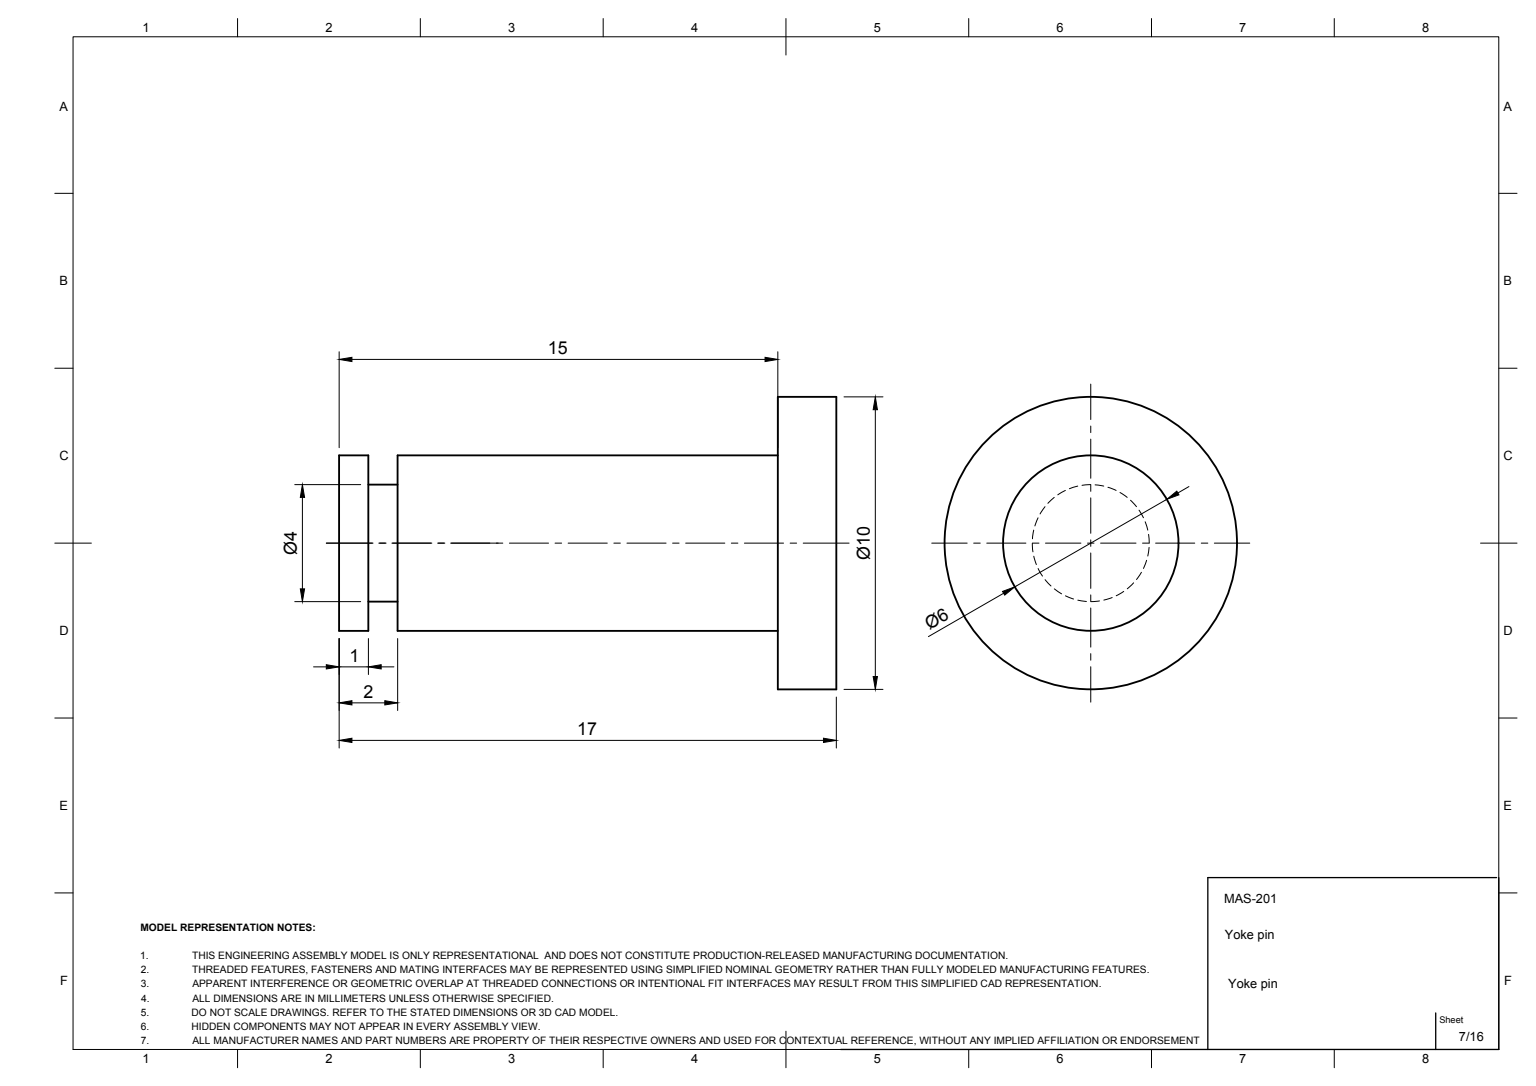
ISO-10303-21;
HEADER;
/* Generated by software containing ST-Developer
 * from STEP Tools, Inc. (www.steptools.com) 
 */

FILE_DESCRIPTION(
/* description */ ('Independent manual two-gate roller-track escapement for nominal30mm d
iameter20mm wide feed rollers. Opposed gates are driven by native capt
ured pin-slot loops with positive curved-slot travel stops at\X\B116de
g. Repeated gate/pin/washer/clip instances, adapted native common bear
ing families, full retaining lips and rotating polymer grip. External 
workpieces, gravity feeder/incline and mount anchors outside assembly.
 No powered-feed compatibility, impact, capacity, safety, force, wear 
or life rating.'),
/* implementation_level */ '2;1');

FILE_NAME(
/* name */ 'Yoke pin.step',
/* time_stamp */ '2026-11-08T18:43:23-08:00',
/* author */ (''),
/* organization */ (''),
/* preprocessor_version */ 'ST-DEVELOPER v20.2',
/* originating_system */ 'Autodesk Translation Framework v15.17.0.0',
/* authorisation */ '');

FILE_SCHEMA (('AUTOMOTIVE_DESIGN { 1 0 10303 214 3 1 1 }'));
ENDSEC;

DATA;
#10=MECHANICAL_DESIGN_GEOMETRIC_PRESENTATION_REPRESENTATION('',(#459),#19863);
#421=SHAPE_REPRESENTATION_RELATIONSHIP('SRR','None',#19939,#440);
#440=ADVANCED_BREP_SHAPE_REPRESENTATION('',(#478),#19848);
#459=STYLED_ITEM('',(#20042),#478);
#478=MANIFOLD_SOLID_BREP('Body1',#6428);
#826=LINE('',#15773,#1291);
#827=LINE('',#15784,#1292);
#828=LINE('',#15792,#1293);
#829=LINE('',#15796,#1294);
#1291=VECTOR('',#8076,2.);
#1292=VECTOR('',#8091,3.);
#1293=VECTOR('',#8100,5.);
#1294=VECTOR('',#8107,3.);
#1536=CYLINDRICAL_SURFACE('',#6927,2.);
#1537=CYLINDRICAL_SURFACE('',#6934,3.);
#1538=CYLINDRICAL_SURFACE('',#6939,5.);
#1539=CYLINDRICAL_SURFACE('',#6942,3.);
#1659=FACE_BOUND('',#2300,.T.);
#1660=FACE_BOUND('',#2302,.T.);
#1661=FACE_BOUND('',#2305,.T.);
#1897=FACE_OUTER_BOUND('',#2298,.T.);
#1898=FACE_OUTER_BOUND('',#2299,.T.);
#1899=FACE_OUTER_BOUND('',#2301,.T.);
#1900=FACE_OUTER_BOUND('',#2303,.T.);
#1901=FACE_OUTER_BOUND('',#2304,.T.);
#1902=FACE_OUTER_BOUND('',#2306,.T.);
#1903=FACE_OUTER_BOUND('',#2307,.T.);
#1904=FACE_OUTER_BOUND('',#2308,.T.);
#1905=FACE_OUTER_BOUND('',#2309,.T.);
#2298=EDGE_LOOP('',(#5289,#5290,#5291,#5292));
#2299=EDGE_LOOP('',(#5293));
#2300=EDGE_LOOP('',(#5294));
#2301=EDGE_LOOP('',(#5295));
#2302=EDGE_LOOP('',(#5296));
#2303=EDGE_LOOP('',(#5297,#5298,#5299,#5300));
#2304=EDGE_LOOP('',(#5301));
#2305=EDGE_LOOP('',(#5302));
#2306=EDGE_LOOP('',(#5303,#5304,#5305,#5306));
#2307=EDGE_LOOP('',(#5307));
#2308=EDGE_LOOP('',(#5308,#5309,#5310,#5311));
#2309=EDGE_LOOP('',(#5312));
#2538=CIRCLE('',#6928,2.);
#2539=CIRCLE('',#6929,2.);
#2540=CIRCLE('',#6931,3.);
#2541=CIRCLE('',#6933,3.);
#2542=CIRCLE('',#6935,3.);
#2543=CIRCLE('',#6937,5.);
#2544=CIRCLE('',#6938,3.);
#2545=CIRCLE('',#6940,5.);
#3008=VERTEX_POINT('',#15770);
#3009=VERTEX_POINT('',#15772);
#3010=VERTEX_POINT('',#15776);
#3011=VERTEX_POINT('',#15779);
#3012=VERTEX_POINT('',#15782);
#3013=VERTEX_POINT('',#15786);
#3014=VERTEX_POINT('',#15788);
#3015=VERTEX_POINT('',#15791);
#3803=EDGE_CURVE('',#3008,#3008,#2538,.T.);
#3804=EDGE_CURVE('',#3008,#3009,#826,.T.);
#3805=EDGE_CURVE('',#3009,#3009,#2539,.T.);
#3806=EDGE_CURVE('',#3010,#3010,#2540,.T.);
#3807=EDGE_CURVE('',#3011,#3011,#2541,.T.);
#3808=EDGE_CURVE('',#3012,#3012,#2542,.T.);
#3809=EDGE_CURVE('',#3012,#3011,#827,.T.);
#3810=EDGE_CURVE('',#3013,#3013,#2543,.T.);
#3811=EDGE_CURVE('',#3014,#3014,#2544,.T.);
#3812=EDGE_CURVE('',#3013,#3015,#828,.T.);
#3813=EDGE_CURVE('',#3015,#3015,#2545,.T.);
#3814=EDGE_CURVE('',#3010,#3014,#829,.T.);
#5289=ORIENTED_EDGE('',*,*,#3803,.T.);
#5290=ORIENTED_EDGE('',*,*,#3804,.T.);
#5291=ORIENTED_EDGE('',*,*,#3805,.F.);
#5292=ORIENTED_EDGE('',*,*,#3804,.F.);
#5293=ORIENTED_EDGE('',*,*,#3806,.F.);
#5294=ORIENTED_EDGE('',*,*,#3803,.F.);
#5295=ORIENTED_EDGE('',*,*,#3807,.F.);
#5296=ORIENTED_EDGE('',*,*,#3805,.T.);
#5297=ORIENTED_EDGE('',*,*,#3808,.F.);
#5298=ORIENTED_EDGE('',*,*,#3809,.T.);
#5299=ORIENTED_EDGE('',*,*,#3807,.T.);
#5300=ORIENTED_EDGE('',*,*,#3809,.F.);
#5301=ORIENTED_EDGE('',*,*,#3810,.T.);
#5302=ORIENTED_EDGE('',*,*,#3811,.F.);
#5303=ORIENTED_EDGE('',*,*,#3810,.F.);
#5304=ORIENTED_EDGE('',*,*,#3812,.T.);
#5305=ORIENTED_EDGE('',*,*,#3813,.T.);
#5306=ORIENTED_EDGE('',*,*,#3812,.F.);
#5307=ORIENTED_EDGE('',*,*,#3813,.F.);
#5308=ORIENTED_EDGE('',*,*,#3806,.T.);
#5309=ORIENTED_EDGE('',*,*,#3814,.T.);
#5310=ORIENTED_EDGE('',*,*,#3811,.T.);
#5311=ORIENTED_EDGE('',*,*,#3814,.F.);
#5312=ORIENTED_EDGE('',*,*,#3808,.T.);
#6004=PLANE('',#6930);
#6005=PLANE('',#6932);
#6006=PLANE('',#6936);
#6007=PLANE('',#6941);
#6008=PLANE('',#6943);
#6276=ADVANCED_FACE('',(#1897),#1536,.T.);
#6277=ADVANCED_FACE('',(#1898,#1659),#6004,.F.);
#6278=ADVANCED_FACE('',(#1899,#1660),#6005,.F.);
#6279=ADVANCED_FACE('',(#1900),#1537,.T.);
#6280=ADVANCED_FACE('',(#1901,#1661),#6006,.T.);
#6281=ADVANCED_FACE('',(#1902),#1538,.T.);
#6282=ADVANCED_FACE('',(#1903),#6007,.F.);
#6283=ADVANCED_FACE('',(#1904),#1539,.T.);
#6284=ADVANCED_FACE('',(#1905),#6008,.T.);
#6428=CLOSED_SHELL('',(#6276,#6277,#6278,#6279,#6280,#6281,#6282,#6283,
#6284));
#6926=AXIS2_PLACEMENT_3D('',#15768,#8070,#8071);
#6927=AXIS2_PLACEMENT_3D('',#15769,#8072,#8073);
#6928=AXIS2_PLACEMENT_3D('',#15771,#8074,#8075);
#6929=AXIS2_PLACEMENT_3D('',#15774,#8077,#8078);
#6930=AXIS2_PLACEMENT_3D('',#15775,#8079,#8080);
#6931=AXIS2_PLACEMENT_3D('',#15777,#8081,#8082);
#6932=AXIS2_PLACEMENT_3D('',#15778,#8083,#8084);
#6933=AXIS2_PLACEMENT_3D('',#15780,#8085,#8086);
#6934=AXIS2_PLACEMENT_3D('',#15781,#8087,#8088);
#6935=AXIS2_PLACEMENT_3D('',#15783,#8089,#8090);
#6936=AXIS2_PLACEMENT_3D('',#15785,#8092,#8093);
#6937=AXIS2_PLACEMENT_3D('',#15787,#8094,#8095);
#6938=AXIS2_PLACEMENT_3D('',#15789,#8096,#8097);
#6939=AXIS2_PLACEMENT_3D('',#15790,#8098,#8099);
#6940=AXIS2_PLACEMENT_3D('',#15793,#8101,#8102);
#6941=AXIS2_PLACEMENT_3D('',#15794,#8103,#8104);
#6942=AXIS2_PLACEMENT_3D('',#15795,#8105,#8106);
#6943=AXIS2_PLACEMENT_3D('',#15797,#8108,#8109);
#8070=DIRECTION('axis',(0.,0.,1.));
#8071=DIRECTION('refdir',(1.,0.,0.));
#8072=DIRECTION('center_axis',(0.,0.,1.));
#8073=DIRECTION('ref_axis',(1.,0.,0.));
#8074=DIRECTION('center_axis',(0.,0.,1.));
#8075=DIRECTION('ref_axis',(1.,0.,0.));
#8076=DIRECTION('',(0.,0.,1.));
#8077=DIRECTION('center_axis',(0.,0.,1.));
#8078=DIRECTION('ref_axis',(1.,0.,0.));
#8079=DIRECTION('center_axis',(0.,0.,-1.));
#8080=DIRECTION('ref_axis',(-1.,0.,0.));
#8081=DIRECTION('center_axis',(0.,0.,-1.));
#8082=DIRECTION('ref_axis',(1.,0.,0.));
#8083=DIRECTION('center_axis',(0.,0.,1.));
#8084=DIRECTION('ref_axis',(1.,0.,0.));
#8085=DIRECTION('center_axis',(0.,0.,1.));
#8086=DIRECTION('ref_axis',(1.,0.,0.));
#8087=DIRECTION('center_axis',(0.,0.,1.));
#8088=DIRECTION('ref_axis',(1.,0.,0.));
#8089=DIRECTION('center_axis',(0.,0.,1.));
#8090=DIRECTION('ref_axis',(1.,0.,0.));
#8091=DIRECTION('',(0.,0.,-1.));
#8092=DIRECTION('center_axis',(0.,0.,1.));
#8093=DIRECTION('ref_axis',(1.,0.,0.));
#8094=DIRECTION('center_axis',(0.,0.,1.));
#8095=DIRECTION('ref_axis',(1.,0.,0.));
#8096=DIRECTION('center_axis',(0.,0.,1.));
#8097=DIRECTION('ref_axis',(1.,0.,0.));
#8098=DIRECTION('center_axis',(0.,0.,1.));
#8099=DIRECTION('ref_axis',(1.,0.,0.));
#8100=DIRECTION('',(0.,0.,-1.));
#8101=DIRECTION('center_axis',(0.,0.,1.));
#8102=DIRECTION('ref_axis',(1.,0.,0.));
#8103=DIRECTION('center_axis',(0.,0.,1.));
#8104=DIRECTION('ref_axis',(1.,0.,0.));
#8105=DIRECTION('center_axis',(0.,0.,1.));
#8106=DIRECTION('ref_axis',(1.,0.,0.));
#8107=DIRECTION('',(0.,0.,-1.));
#8108=DIRECTION('center_axis',(0.,0.,1.));
#8109=DIRECTION('ref_axis',(1.,0.,0.));
#15768=CARTESIAN_POINT('',(0.,0.,0.));
#15769=CARTESIAN_POINT('Origin',(0.,0.,13.5));
#15770=CARTESIAN_POINT('',(-2.,-2.44929359829471E-16,13.));
#15771=CARTESIAN_POINT('Origin',(0.,0.,13.));
#15772=CARTESIAN_POINT('',(-2.,-2.44929359829471E-16,14.));
#15773=CARTESIAN_POINT('',(-2.,-2.44929359829471E-16,13.5));
#15774=CARTESIAN_POINT('Origin',(0.,0.,14.));
#15775=CARTESIAN_POINT('Origin',(6.,0.,13.));
#15776=CARTESIAN_POINT('',(-3.,3.67394039744206E-16,13.));
#15777=CARTESIAN_POINT('Origin',(0.,0.,13.));
#15778=CARTESIAN_POINT('Origin',(2.,0.,14.));
#15779=CARTESIAN_POINT('',(-3.,-3.67394039744206E-16,14.));
#15780=CARTESIAN_POINT('Origin',(0.,0.,14.));
#15781=CARTESIAN_POINT('Origin',(0.,0.,0.));
#15782=CARTESIAN_POINT('',(-3.,-3.67394039744206E-16,15.));
#15783=CARTESIAN_POINT('Origin',(0.,0.,15.));
#15784=CARTESIAN_POINT('',(-3.,-3.67394039744206E-16,0.));
#15785=CARTESIAN_POINT('Origin',(0.,0.,0.));
#15786=CARTESIAN_POINT('',(-5.,-6.12323399573677E-16,0.));
#15787=CARTESIAN_POINT('Origin',(0.,0.,0.));
#15788=CARTESIAN_POINT('',(-3.,-3.67394039744206E-16,0.));
#15789=CARTESIAN_POINT('Origin',(0.,0.,0.));
#15790=CARTESIAN_POINT('Origin',(0.,0.,-2.));
#15791=CARTESIAN_POINT('',(-5.,-6.12323399573677E-16,-2.));
#15792=CARTESIAN_POINT('',(-5.,-6.12323399573677E-16,-2.));
#15793=CARTESIAN_POINT('Origin',(0.,0.,-2.));
#15794=CARTESIAN_POINT('Origin',(0.,0.,-2.));
#15795=CARTESIAN_POINT('Origin',(0.,0.,0.));
#15796=CARTESIAN_POINT('',(-3.,-3.67394039744206E-16,0.));
#15797=CARTESIAN_POINT('Origin',(0.,0.,15.));
#19827=UNCERTAINTY_MEASURE_WITH_UNIT(LENGTH_MEASURE(0.01),#19864,
'DISTANCE_ACCURACY_VALUE',
'Maximum model space distance between geometric entities at asserted c
onnectivities');
#19842=UNCERTAINTY_MEASURE_WITH_UNIT(LENGTH_MEASURE(0.01),#19864,
'DISTANCE_ACCURACY_VALUE',
'Maximum model space distance between geometric entities at asserted c
onnectivities');
#19848=(
GEOMETRIC_REPRESENTATION_CONTEXT(3)
GLOBAL_UNCERTAINTY_ASSIGNED_CONTEXT((#19827))
GLOBAL_UNIT_ASSIGNED_CONTEXT((#19864,#19866,#19867))
REPRESENTATION_CONTEXT('','3D')
);
#19863=(
GEOMETRIC_REPRESENTATION_CONTEXT(3)
GLOBAL_UNCERTAINTY_ASSIGNED_CONTEXT((#19842))
GLOBAL_UNIT_ASSIGNED_CONTEXT((#19864,#19866,#19867))
REPRESENTATION_CONTEXT('','3D')
);
#19864=(
LENGTH_UNIT()
NAMED_UNIT(*)
SI_UNIT(.MILLI.,.METRE.)
);
#19866=(
NAMED_UNIT(*)
PLANE_ANGLE_UNIT()
SI_UNIT($,.RADIAN.)
);
#19867=(
NAMED_UNIT(*)
SI_UNIT($,.STERADIAN.)
SOLID_ANGLE_UNIT()
);
#19873=SHAPE_DEFINITION_REPRESENTATION(#19893,#19939);
#19893=PRODUCT_DEFINITION_SHAPE('',$,#19960);
#19939=SHAPE_REPRESENTATION('',(#6926),#19848);
#19954=PRODUCT_DEFINITION_CONTEXT('part definition',#20016,'design');
#19960=PRODUCT_DEFINITION('Yoke pin','Yoke pin',#19980,#19954);
#19980=PRODUCT_DEFINITION_FORMATION('',$,#20023);
#20016=APPLICATION_CONTEXT(
'Core Data for Automotive Mechanical Design Process');
#20017=PRODUCT_CONTEXT('part definition',#20016,'mechanical');
#20023=PRODUCT('Yoke pin','Yoke pin',$,(#20017));
#20042=PRESENTATION_STYLE_ASSIGNMENT((#20049));
#20049=SURFACE_STYLE_USAGE(.BOTH.,#20056);
#20056=SURFACE_SIDE_STYLE('',(#20063));
#20063=SURFACE_STYLE_FILL_AREA(#20070);
#20070=FILL_AREA_STYLE('Gray',(#20077));
#20077=FILL_AREA_STYLE_COLOUR('Gray',#20084);
#20084=COLOUR_RGB('Gray',0.407843137254902,0.447058823529412,0.498039215686275);
ENDSEC;
END-ISO-10303-21;
